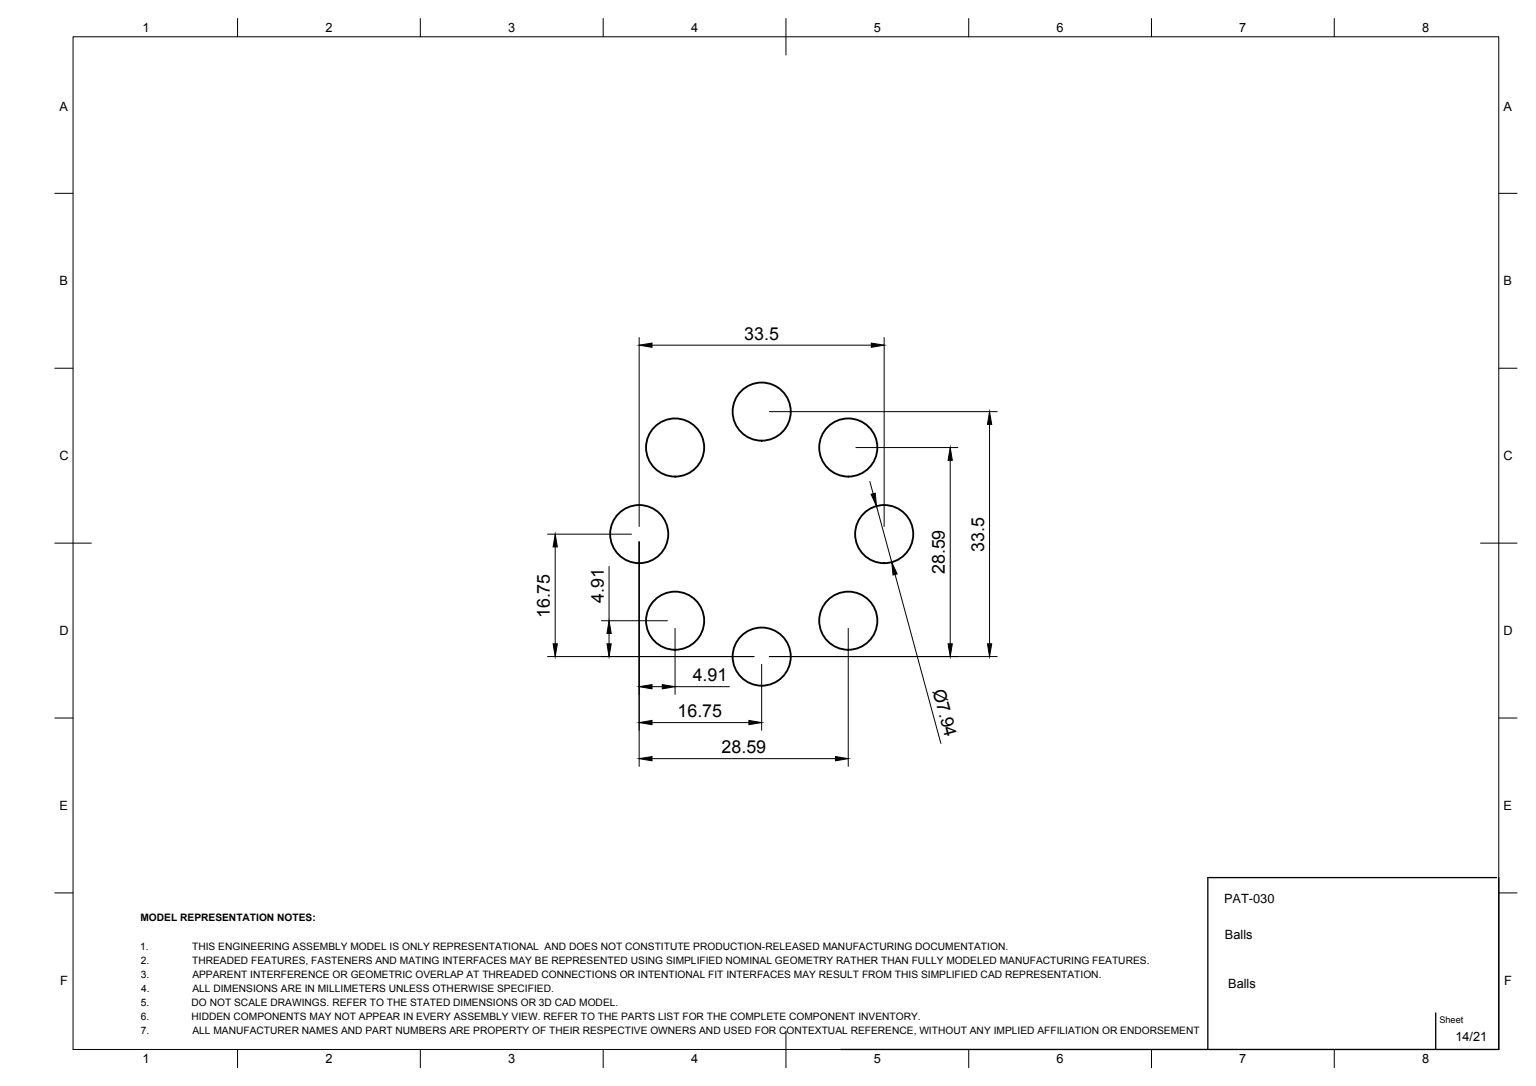
ISO-10303-21;
HEADER;
/* Generated by software containing ST-Developer
 * from STEP Tools, Inc. (www.steptools.com) 
 */

FILE_DESCRIPTION(
/* description */ ('Double-bearing flanged cartridge'),
/* implementation_level */ '2;1');

FILE_NAME(
/* name */ 'Balls.step',
/* time_stamp */ '2026-10-28T03:26:40-07:00',
/* author */ (''),
/* organization */ (''),
/* preprocessor_version */ 'ST-DEVELOPER v20.2',
/* originating_system */ 'Autodesk Translation Framework v15.17.0.0',
/* authorisation */ '');

FILE_SCHEMA (('AUTOMOTIVE_DESIGN { 1 0 10303 214 3 1 1 }'));
ENDSEC;

DATA;
#10=MECHANICAL_DESIGN_GEOMETRIC_PRESENTATION_REPRESENTATION('',(#193,#194,#195,#196,#197,#198,#199,#200),#5535);
#136=SPHERICAL_SURFACE('',#2607,0.3969);
#137=SPHERICAL_SURFACE('',#2609,0.3969);
#138=SPHERICAL_SURFACE('',#2611,0.3969);
#139=SPHERICAL_SURFACE('',#2613,0.3969);
#140=SPHERICAL_SURFACE('',#2615,0.3969);
#141=SPHERICAL_SURFACE('',#2617,0.3969);
#142=SPHERICAL_SURFACE('',#2619,0.3969);
#143=SPHERICAL_SURFACE('',#2621,0.3969);
#165=SHAPE_REPRESENTATION_RELATIONSHIP('SRR','None',#5607,#179);
#179=ADVANCED_BREP_SHAPE_REPRESENTATION('',(#215,#216,#217,#218,#219,#220,
#221,#222),#5523);
#193=STYLED_ITEM('',(#5764),#215);
#194=STYLED_ITEM('',(#5764),#216);
#195=STYLED_ITEM('',(#5764),#217);
#196=STYLED_ITEM('',(#5764),#218);
#197=STYLED_ITEM('',(#5764),#219);
#198=STYLED_ITEM('',(#5764),#220);
#199=STYLED_ITEM('',(#5764),#221);
#200=STYLED_ITEM('',(#5764),#222);
#215=MANIFOLD_SOLID_BREP('Body1',#2327);
#216=MANIFOLD_SOLID_BREP('Body2',#2328);
#217=MANIFOLD_SOLID_BREP('Body3',#2329);
#218=MANIFOLD_SOLID_BREP('Body4',#2330);
#219=MANIFOLD_SOLID_BREP('Body5',#2331);
#220=MANIFOLD_SOLID_BREP('Body6',#2332);
#221=MANIFOLD_SOLID_BREP('Body7',#2333);
#222=MANIFOLD_SOLID_BREP('Body8',#2334);
#405=FACE_OUTER_BOUND('',#578,.T.);
#406=FACE_OUTER_BOUND('',#579,.T.);
#407=FACE_OUTER_BOUND('',#580,.T.);
#408=FACE_OUTER_BOUND('',#581,.T.);
#409=FACE_OUTER_BOUND('',#582,.T.);
#410=FACE_OUTER_BOUND('',#583,.T.);
#411=FACE_OUTER_BOUND('',#584,.T.);
#412=FACE_OUTER_BOUND('',#585,.T.);
#578=EDGE_LOOP('',(#1710,#1711));
#579=EDGE_LOOP('',(#1712,#1713));
#580=EDGE_LOOP('',(#1714,#1715));
#581=EDGE_LOOP('',(#1716,#1717));
#582=EDGE_LOOP('',(#1718,#1719));
#583=EDGE_LOOP('',(#1720,#1721));
#584=EDGE_LOOP('',(#1722,#1723));
#585=EDGE_LOOP('',(#1724,#1725));
#952=CIRCLE('',#2608,0.3969);
#953=CIRCLE('',#2610,0.3969);
#954=CIRCLE('',#2612,0.3969);
#955=CIRCLE('',#2614,0.3969);
#956=CIRCLE('',#2616,0.3969);
#957=CIRCLE('',#2618,0.3969);
#958=CIRCLE('',#2620,0.3969);
#959=CIRCLE('',#2622,0.3969);
#1124=VERTEX_POINT('',#3867);
#1125=VERTEX_POINT('',#3868);
#1126=VERTEX_POINT('',#3871);
#1127=VERTEX_POINT('',#3872);
#1128=VERTEX_POINT('',#3875);
#1129=VERTEX_POINT('',#3876);
#1130=VERTEX_POINT('',#3879);
#1131=VERTEX_POINT('',#3880);
#1132=VERTEX_POINT('',#3883);
#1133=VERTEX_POINT('',#3884);
#1134=VERTEX_POINT('',#3887);
#1135=VERTEX_POINT('',#3888);
#1136=VERTEX_POINT('',#3891);
#1137=VERTEX_POINT('',#3892);
#1138=VERTEX_POINT('',#3895);
#1139=VERTEX_POINT('',#3896);
#1348=EDGE_CURVE('',#1124,#1125,#952,.T.);
#1349=EDGE_CURVE('',#1126,#1127,#953,.T.);
#1350=EDGE_CURVE('',#1128,#1129,#954,.T.);
#1351=EDGE_CURVE('',#1130,#1131,#955,.T.);
#1352=EDGE_CURVE('',#1132,#1133,#956,.T.);
#1353=EDGE_CURVE('',#1134,#1135,#957,.T.);
#1354=EDGE_CURVE('',#1136,#1137,#958,.T.);
#1355=EDGE_CURVE('',#1138,#1139,#959,.T.);
#1710=ORIENTED_EDGE('',*,*,#1348,.T.);
#1711=ORIENTED_EDGE('',*,*,#1348,.F.);
#1712=ORIENTED_EDGE('',*,*,#1349,.T.);
#1713=ORIENTED_EDGE('',*,*,#1349,.F.);
#1714=ORIENTED_EDGE('',*,*,#1350,.T.);
#1715=ORIENTED_EDGE('',*,*,#1350,.F.);
#1716=ORIENTED_EDGE('',*,*,#1351,.T.);
#1717=ORIENTED_EDGE('',*,*,#1351,.F.);
#1718=ORIENTED_EDGE('',*,*,#1352,.T.);
#1719=ORIENTED_EDGE('',*,*,#1352,.F.);
#1720=ORIENTED_EDGE('',*,*,#1353,.T.);
#1721=ORIENTED_EDGE('',*,*,#1353,.F.);
#1722=ORIENTED_EDGE('',*,*,#1354,.T.);
#1723=ORIENTED_EDGE('',*,*,#1354,.F.);
#1724=ORIENTED_EDGE('',*,*,#1355,.T.);
#1725=ORIENTED_EDGE('',*,*,#1355,.F.);
#2219=ADVANCED_FACE('',(#405),#136,.T.);
#2220=ADVANCED_FACE('',(#406),#137,.T.);
#2221=ADVANCED_FACE('',(#407),#138,.T.);
#2222=ADVANCED_FACE('',(#408),#139,.T.);
#2223=ADVANCED_FACE('',(#409),#140,.T.);
#2224=ADVANCED_FACE('',(#410),#141,.T.);
#2225=ADVANCED_FACE('',(#411),#142,.T.);
#2226=ADVANCED_FACE('',(#412),#143,.T.);
#2327=CLOSED_SHELL('',(#2219));
#2328=CLOSED_SHELL('',(#2220));
#2329=CLOSED_SHELL('',(#2221));
#2330=CLOSED_SHELL('',(#2222));
#2331=CLOSED_SHELL('',(#2223));
#2332=CLOSED_SHELL('',(#2224));
#2333=CLOSED_SHELL('',(#2225));
#2334=CLOSED_SHELL('',(#2226));
#2606=AXIS2_PLACEMENT_3D('',#3865,#3101,#3102);
#2607=AXIS2_PLACEMENT_3D('',#3866,#3103,#3104);
#2608=AXIS2_PLACEMENT_3D('',#3869,#3105,#3106);
#2609=AXIS2_PLACEMENT_3D('',#3870,#3107,#3108);
#2610=AXIS2_PLACEMENT_3D('',#3873,#3109,#3110);
#2611=AXIS2_PLACEMENT_3D('',#3874,#3111,#3112);
#2612=AXIS2_PLACEMENT_3D('',#3877,#3113,#3114);
#2613=AXIS2_PLACEMENT_3D('',#3878,#3115,#3116);
#2614=AXIS2_PLACEMENT_3D('',#3881,#3117,#3118);
#2615=AXIS2_PLACEMENT_3D('',#3882,#3119,#3120);
#2616=AXIS2_PLACEMENT_3D('',#3885,#3121,#3122);
#2617=AXIS2_PLACEMENT_3D('',#3886,#3123,#3124);
#2618=AXIS2_PLACEMENT_3D('',#3889,#3125,#3126);
#2619=AXIS2_PLACEMENT_3D('',#3890,#3127,#3128);
#2620=AXIS2_PLACEMENT_3D('',#3893,#3129,#3130);
#2621=AXIS2_PLACEMENT_3D('',#3894,#3131,#3132);
#2622=AXIS2_PLACEMENT_3D('',#3897,#3133,#3134);
#3101=DIRECTION('axis',(0.,0.,1.));
#3102=DIRECTION('refdir',(1.,0.,0.));
#3103=DIRECTION('center_axis',(0.,0.,1.));
#3104=DIRECTION('ref_axis',(1.,0.,0.));
#3105=DIRECTION('center_axis',(1.22464679914735E-16,-1.,0.));
#3106=DIRECTION('ref_axis',(-1.,-1.22464679914735E-16,0.));
#3107=DIRECTION('center_axis',(0.707106781186548,0.,0.707106781186548));
#3108=DIRECTION('ref_axis',(0.707106781186548,0.,-0.707106781186548));
#3109=DIRECTION('center_axis',(8.65956056235493E-17,-1.,-8.65956056235493E-17));
#3110=DIRECTION('ref_axis',(-0.707106781186548,-1.22464679914735E-16,0.707106781186548));
#3111=DIRECTION('center_axis',(1.,0.,0.));
#3112=DIRECTION('ref_axis',(6.12323399573677E-17,0.,-1.));
#3113=DIRECTION('center_axis',(7.49879891330929E-33,-1.,-1.22464679914735E-16));
#3114=DIRECTION('ref_axis',(-6.12323399573677E-17,-1.22464679914735E-16,
1.));
#3115=DIRECTION('center_axis',(0.707106781186548,0.,-0.707106781186548));
#3116=DIRECTION('ref_axis',(-0.707106781186548,0.,-0.707106781186548));
#3117=DIRECTION('center_axis',(-8.65956056235493E-17,-1.,-8.65956056235493E-17));
#3118=DIRECTION('ref_axis',(0.707106781186548,-1.22464679914735E-16,0.707106781186548));
#3119=DIRECTION('center_axis',(0.,0.,-1.));
#3120=DIRECTION('ref_axis',(-1.,0.,-1.22464679914735E-16));
#3121=DIRECTION('center_axis',(-1.22464679914735E-16,-1.,-1.49975978266186E-32));
#3122=DIRECTION('ref_axis',(1.,-1.22464679914735E-16,1.22464679914735E-16));
#3123=DIRECTION('center_axis',(-0.707106781186548,0.,-0.707106781186548));
#3124=DIRECTION('ref_axis',(-0.707106781186548,0.,0.707106781186548));
#3125=DIRECTION('center_axis',(-8.65956056235493E-17,-1.,8.65956056235493E-17));
#3126=DIRECTION('ref_axis',(0.707106781186548,-1.22464679914735E-16,-0.707106781186548));
#3127=DIRECTION('center_axis',(-1.,0.,0.));
#3128=DIRECTION('ref_axis',(-1.83697019872103E-16,0.,1.));
#3129=DIRECTION('center_axis',(-2.24963967399279E-32,-1.,1.22464679914735E-16));
#3130=DIRECTION('ref_axis',(1.83697019872103E-16,-1.22464679914735E-16,
-1.));
#3131=DIRECTION('center_axis',(-0.707106781186548,0.,0.707106781186548));
#3132=DIRECTION('ref_axis',(0.707106781186548,0.,0.707106781186548));
#3133=DIRECTION('center_axis',(8.65956056235493E-17,-1.,8.65956056235494E-17));
#3134=DIRECTION('ref_axis',(-0.707106781186548,-1.22464679914735E-16,-0.707106781186548));
#3865=CARTESIAN_POINT('',(0.,0.,0.));
#3866=CARTESIAN_POINT('Origin',(1.675,0.,0.));
#3867=CARTESIAN_POINT('',(1.675,-2.97627328869245E-33,0.3969));
#3868=CARTESIAN_POINT('',(1.675,-2.97627328869245E-33,-0.3969));
#3869=CARTESIAN_POINT('Origin',(1.675,0.,0.));
#3870=CARTESIAN_POINT('Origin',(1.18440385848747,0.,-1.18440385848747));
#3871=CARTESIAN_POINT('',(1.46505453994041,3.1867025333467E-33,-0.903753177034526));
#3872=CARTESIAN_POINT('',(0.903753177034527,-9.13924911073161E-33,-1.46505453994041));
#3873=CARTESIAN_POINT('Origin',(1.18440385848747,0.,-1.18440385848747));
#3874=CARTESIAN_POINT('Origin',(1.02564169428591E-16,0.,-1.675));
#3875=CARTESIAN_POINT('',(0.3969,-2.97627328869246E-33,-1.675));
#3876=CARTESIAN_POINT('',(-0.3969,-2.97627328869245E-33,-1.675));
#3877=CARTESIAN_POINT('Origin',(1.02564169428591E-16,0.,-1.675));
#3878=CARTESIAN_POINT('Origin',(-1.18440385848747,0.,-1.18440385848747));
#3879=CARTESIAN_POINT('',(-0.903753177034526,3.1867025333467E-33,-1.46505453994041));
#3880=CARTESIAN_POINT('',(-1.46505453994041,-9.13924911073161E-33,-0.903753177034527));
#3881=CARTESIAN_POINT('Origin',(-1.18440385848747,0.,-1.18440385848747));
#3882=CARTESIAN_POINT('Origin',(-1.675,0.,-2.05128338857182E-16));
#3883=CARTESIAN_POINT('',(-1.675,-2.97627328869246E-33,-0.3969));
#3884=CARTESIAN_POINT('',(-1.675,-2.97627328869245E-33,0.3969));
#3885=CARTESIAN_POINT('Origin',(-1.675,0.,-2.05128338857182E-16));
#3886=CARTESIAN_POINT('Origin',(-1.18440385848747,0.,1.18440385848747));
#3887=CARTESIAN_POINT('',(-1.46505453994041,6.26819044436628E-33,0.903753177034526));
#3888=CARTESIAN_POINT('',(-0.903753177034527,-1.22207370217512E-32,1.46505453994041));
#3889=CARTESIAN_POINT('Origin',(-1.18440385848747,0.,1.18440385848747));
#3890=CARTESIAN_POINT('Origin',(-3.07692508285772E-16,0.,1.675));
#3891=CARTESIAN_POINT('',(-0.3969,-2.97627328869246E-33,1.675));
#3892=CARTESIAN_POINT('',(0.396899999999999,-2.97627328869245E-33,1.675));
#3893=CARTESIAN_POINT('Origin',(-3.07692508285772E-16,0.,1.675));
#3894=CARTESIAN_POINT('Origin',(1.18440385848747,0.,1.18440385848747));
#3895=CARTESIAN_POINT('',(0.903753177034526,9.34967835538585E-33,1.46505453994041));
#3896=CARTESIAN_POINT('',(1.46505453994041,-1.53022249327708E-32,0.903753177034527));
#3897=CARTESIAN_POINT('Origin',(1.18440385848747,0.,1.18440385848747));
#5504=UNCERTAINTY_MEASURE_WITH_UNIT(LENGTH_MEASURE(0.001),#5536,
'DISTANCE_ACCURACY_VALUE',
'Maximum model space distance between geometric entities at asserted c
onnectivities');
#5516=UNCERTAINTY_MEASURE_WITH_UNIT(LENGTH_MEASURE(0.001),#5536,
'DISTANCE_ACCURACY_VALUE',
'Maximum model space distance between geometric entities at asserted c
onnectivities');
#5523=(
GEOMETRIC_REPRESENTATION_CONTEXT(3)
GLOBAL_UNCERTAINTY_ASSIGNED_CONTEXT((#5504))
GLOBAL_UNIT_ASSIGNED_CONTEXT((#5536,#5538,#5539))
REPRESENTATION_CONTEXT('','3D')
);
#5535=(
GEOMETRIC_REPRESENTATION_CONTEXT(3)
GLOBAL_UNCERTAINTY_ASSIGNED_CONTEXT((#5516))
GLOBAL_UNIT_ASSIGNED_CONTEXT((#5536,#5538,#5539))
REPRESENTATION_CONTEXT('','3D')
);
#5536=(
LENGTH_UNIT()
NAMED_UNIT(*)
SI_UNIT(.CENTI.,.METRE.)
);
#5538=(
NAMED_UNIT(*)
PLANE_ANGLE_UNIT()
SI_UNIT($,.RADIAN.)
);
#5539=(
NAMED_UNIT(*)
SI_UNIT($,.STERADIAN.)
SOLID_ANGLE_UNIT()
);
#5546=SHAPE_DEFINITION_REPRESENTATION(#5564,#5607);
#5564=PRODUCT_DEFINITION_SHAPE('',$,#5626);
#5607=SHAPE_REPRESENTATION('',(#2606),#5523);
#5619=PRODUCT_DEFINITION_CONTEXT('part definition',#5675,'design');
#5626=PRODUCT_DEFINITION('Balls','Balls',#5644,#5619);
#5644=PRODUCT_DEFINITION_FORMATION('',$,#5683);
#5675=APPLICATION_CONTEXT(
'Core Data for Automotive Mechanical Design Process');
#5676=PRODUCT_CONTEXT('part definition',#5675,'mechanical');
#5683=PRODUCT('Balls','Balls','Balls',(#5676));
#5758=COLOUR_RGB('Grey',0.48,0.52,0.57);
#5759=FILL_AREA_STYLE_COLOUR('',#5758);
#5760=FILL_AREA_STYLE('',(#5759));
#5761=SURFACE_STYLE_FILL_AREA(#5760);
#5762=SURFACE_SIDE_STYLE('',(#5761));
#5763=SURFACE_STYLE_USAGE(.BOTH.,#5762);
#5764=PRESENTATION_STYLE_ASSIGNMENT((#5763));
ENDSEC;
END-ISO-10303-21;
